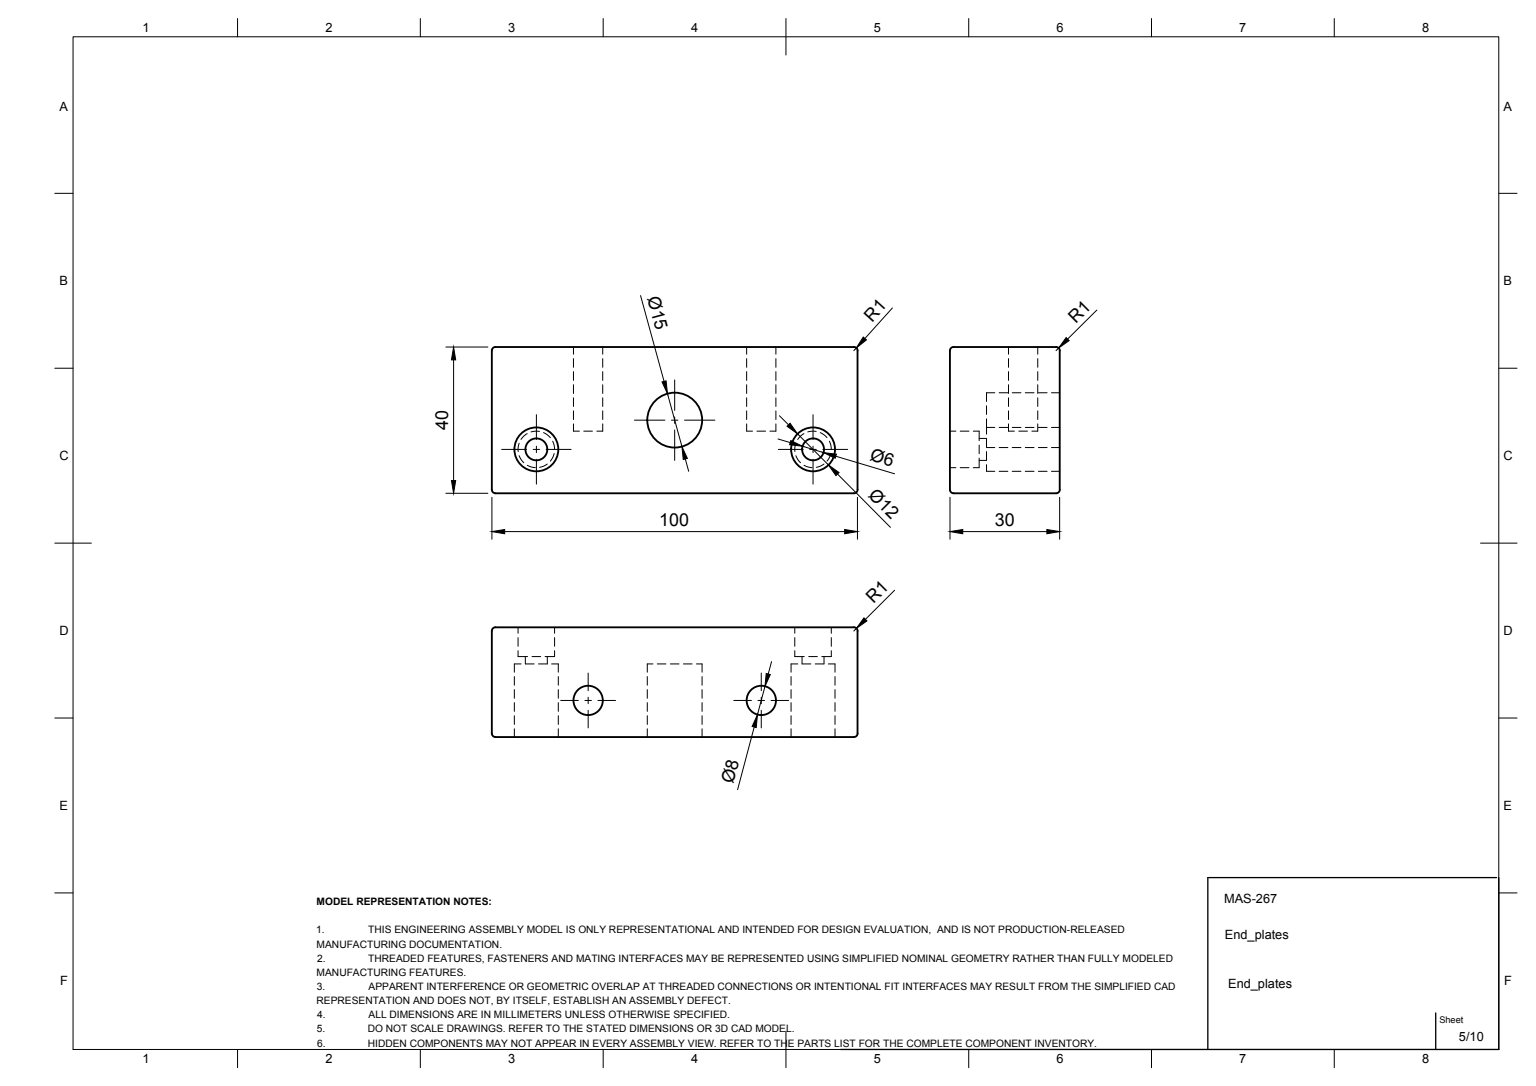
ISO-10303-21;
HEADER;
/* Generated by software containing ST-Developer
 * from STEP Tools, Inc. (www.steptools.com) 
 */

FILE_DESCRIPTION(
/* description */ (''),
/* implementation_level */ '2;1');

FILE_NAME(
/* name */ 'End_plates.step',
/* time_stamp */ '2026-10-12T15:29:24-07:00',
/* author */ (''),
/* organization */ (''),
/* preprocessor_version */ 'ST-DEVELOPER v20.2',
/* originating_system */ 'Autodesk Translation Framework v15.15.0.0',
/* authorisation */ '');

FILE_SCHEMA (('AUTOMOTIVE_DESIGN { 1 0 10303 214 3 1 1 }'));
ENDSEC;

DATA;
#10=MECHANICAL_DESIGN_GEOMETRIC_PRESENTATION_REPRESENTATION('',(#164),#9496);
#146=SHAPE_REPRESENTATION_RELATIONSHIP('SRR','None',#9540,#155);
#155=ADVANCED_BREP_SHAPE_REPRESENTATION('',(#221),#9488);
#164=STYLED_ITEM('',(#9593),#221);
#221=MANIFOLD_SOLID_BREP('Body1',#4966);
#285=SPHERICAL_SURFACE('',#5240,0.999999999999996);
#286=SPHERICAL_SURFACE('',#5244,1.00000000000001);
#287=SPHERICAL_SURFACE('',#5248,1.00000000000001);
#288=SPHERICAL_SURFACE('',#5252,0.999999999999996);
#289=SPHERICAL_SURFACE('',#5257,0.999999999999996);
#290=SPHERICAL_SURFACE('',#5261,0.999999999999996);
#291=SPHERICAL_SURFACE('',#5266,0.999999999999996);
#292=SPHERICAL_SURFACE('',#5272,1.00000000000001);
#343=FACE_BOUND('',#1011,.T.);
#344=FACE_BOUND('',#1018,.T.);
#345=FACE_BOUND('',#1021,.T.);
#346=FACE_BOUND('',#1045,.T.);
#347=FACE_BOUND('',#1046,.T.);
#348=FACE_BOUND('',#1047,.T.);
#349=FACE_BOUND('',#1050,.T.);
#350=FACE_BOUND('',#1051,.T.);
#351=FACE_BOUND('',#1054,.T.);
#352=FACE_BOUND('',#1055,.T.);
#353=FACE_BOUND('',#1059,.T.);
#498=PLANE('',#5217);
#499=PLANE('',#5222);
#500=PLANE('',#5226);
#501=PLANE('',#5230);
#502=PLANE('',#5235);
#503=PLANE('',#5284);
#504=PLANE('',#5287);
#505=PLANE('',#5288);
#506=PLANE('',#5289);
#507=PLANE('',#5290);
#508=PLANE('',#5291);
#509=PLANE('',#5294);
#510=PLANE('',#5297);
#667=FACE_OUTER_BOUND('',#1009,.T.);
#668=FACE_OUTER_BOUND('',#1010,.T.);
#669=FACE_OUTER_BOUND('',#1012,.T.);
#670=FACE_OUTER_BOUND('',#1013,.T.);
#671=FACE_OUTER_BOUND('',#1014,.T.);
#672=FACE_OUTER_BOUND('',#1015,.T.);
#673=FACE_OUTER_BOUND('',#1016,.T.);
#674=FACE_OUTER_BOUND('',#1017,.T.);
#675=FACE_OUTER_BOUND('',#1019,.T.);
#676=FACE_OUTER_BOUND('',#1020,.T.);
#677=FACE_OUTER_BOUND('',#1022,.T.);
#678=FACE_OUTER_BOUND('',#1023,.T.);
#679=FACE_OUTER_BOUND('',#1024,.T.);
#680=FACE_OUTER_BOUND('',#1025,.T.);
#681=FACE_OUTER_BOUND('',#1026,.T.);
#682=FACE_OUTER_BOUND('',#1027,.T.);
#683=FACE_OUTER_BOUND('',#1028,.T.);
#684=FACE_OUTER_BOUND('',#1029,.T.);
#685=FACE_OUTER_BOUND('',#1030,.T.);
#686=FACE_OUTER_BOUND('',#1031,.T.);
#687=FACE_OUTER_BOUND('',#1032,.T.);
#688=FACE_OUTER_BOUND('',#1033,.T.);
#689=FACE_OUTER_BOUND('',#1034,.T.);
#690=FACE_OUTER_BOUND('',#1035,.T.);
#691=FACE_OUTER_BOUND('',#1036,.T.);
#692=FACE_OUTER_BOUND('',#1037,.T.);
#693=FACE_OUTER_BOUND('',#1038,.T.);
#694=FACE_OUTER_BOUND('',#1039,.T.);
#695=FACE_OUTER_BOUND('',#1040,.T.);
#696=FACE_OUTER_BOUND('',#1041,.T.);
#697=FACE_OUTER_BOUND('',#1042,.T.);
#698=FACE_OUTER_BOUND('',#1043,.T.);
#699=FACE_OUTER_BOUND('',#1044,.T.);
#700=FACE_OUTER_BOUND('',#1048,.T.);
#701=FACE_OUTER_BOUND('',#1049,.T.);
#702=FACE_OUTER_BOUND('',#1052,.T.);
#703=FACE_OUTER_BOUND('',#1053,.T.);
#704=FACE_OUTER_BOUND('',#1056,.T.);
#705=FACE_OUTER_BOUND('',#1057,.T.);
#706=FACE_OUTER_BOUND('',#1058,.T.);
#707=FACE_OUTER_BOUND('',#1060,.T.);
#708=FACE_OUTER_BOUND('',#1061,.T.);
#1009=EDGE_LOOP('',(#3507,#3508,#3509,#3510));
#1010=EDGE_LOOP('',(#3511));
#1011=EDGE_LOOP('',(#3512));
#1012=EDGE_LOOP('',(#3513,#3514,#3515,#3516));
#1013=EDGE_LOOP('',(#3517));
#1014=EDGE_LOOP('',(#3518,#3519,#3520,#3521));
#1015=EDGE_LOOP('',(#3522));
#1016=EDGE_LOOP('',(#3523,#3524,#3525,#3526));
#1017=EDGE_LOOP('',(#3527));
#1018=EDGE_LOOP('',(#3528));
#1019=EDGE_LOOP('',(#3529,#3530,#3531,#3532));
#1020=EDGE_LOOP('',(#3533));
#1021=EDGE_LOOP('',(#3534));
#1022=EDGE_LOOP('',(#3535,#3536,#3537,#3538));
#1023=EDGE_LOOP('',(#3539,#3540,#3541,#3542));
#1024=EDGE_LOOP('',(#3543,#3544,#3545));
#1025=EDGE_LOOP('',(#3546,#3547,#3548));
#1026=EDGE_LOOP('',(#3549,#3550,#3551));
#1027=EDGE_LOOP('',(#3552,#3553,#3554));
#1028=EDGE_LOOP('',(#3555,#3556,#3557,#3558));
#1029=EDGE_LOOP('',(#3559,#3560,#3561));
#1030=EDGE_LOOP('',(#3562,#3563,#3564));
#1031=EDGE_LOOP('',(#3565,#3566,#3567,#3568));
#1032=EDGE_LOOP('',(#3569,#3570,#3571));
#1033=EDGE_LOOP('',(#3572,#3573,#3574,#3575));
#1034=EDGE_LOOP('',(#3576,#3577,#3578,#3579));
#1035=EDGE_LOOP('',(#3580,#3581,#3582));
#1036=EDGE_LOOP('',(#3583,#3584,#3585,#3586));
#1037=EDGE_LOOP('',(#3587,#3588,#3589,#3590));
#1038=EDGE_LOOP('',(#3591,#3592,#3593,#3594));
#1039=EDGE_LOOP('',(#3595,#3596,#3597,#3598));
#1040=EDGE_LOOP('',(#3599,#3600,#3601,#3602));
#1041=EDGE_LOOP('',(#3603,#3604,#3605,#3606));
#1042=EDGE_LOOP('',(#3607,#3608,#3609,#3610));
#1043=EDGE_LOOP('',(#3611,#3612,#3613,#3614));
#1044=EDGE_LOOP('',(#3615,#3616,#3617,#3618));
#1045=EDGE_LOOP('',(#3619));
#1046=EDGE_LOOP('',(#3620));
#1047=EDGE_LOOP('',(#3621));
#1048=EDGE_LOOP('',(#3622,#3623,#3624,#3625));
#1049=EDGE_LOOP('',(#3626,#3627,#3628,#3629));
#1050=EDGE_LOOP('',(#3630));
#1051=EDGE_LOOP('',(#3631));
#1052=EDGE_LOOP('',(#3632,#3633,#3634,#3635));
#1053=EDGE_LOOP('',(#3636,#3637,#3638,#3639));
#1054=EDGE_LOOP('',(#3640));
#1055=EDGE_LOOP('',(#3641));
#1056=EDGE_LOOP('',(#3642,#3643,#3644,#3645));
#1057=EDGE_LOOP('',(#3646,#3647,#3648,#3649));
#1058=EDGE_LOOP('',(#3650));
#1059=EDGE_LOOP('',(#3651));
#1060=EDGE_LOOP('',(#3652,#3653,#3654,#3655));
#1061=EDGE_LOOP('',(#3656));
#1482=LINE('',#7668,#1719);
#1483=LINE('',#7677,#1720);
#1484=LINE('',#7684,#1721);
#1485=LINE('',#7691,#1722);
#1486=LINE('',#7700,#1723);
#1487=LINE('',#7706,#1724);
#1488=LINE('',#7709,#1725);
#1489=LINE('',#7740,#1726);
#1490=LINE('',#7741,#1727);
#1491=LINE('',#7757,#1728);
#1492=LINE('',#7758,#1729);
#1493=LINE('',#7767,#1730);
#1494=LINE('',#7768,#1731);
#1495=LINE('',#7770,#1732);
#1496=LINE('',#7771,#1733);
#1497=LINE('',#7780,#1734);
#1498=LINE('',#7781,#1735);
#1499=LINE('',#7783,#1736);
#1500=LINE('',#7784,#1737);
#1501=LINE('',#7786,#1738);
#1502=LINE('',#7787,#1739);
#1503=LINE('',#7789,#1740);
#1504=LINE('',#7790,#1741);
#1505=LINE('',#7792,#1742);
#1506=LINE('',#7793,#1743);
#1507=LINE('',#7795,#1744);
#1508=LINE('',#7796,#1745);
#1509=LINE('',#7798,#1746);
#1510=LINE('',#7799,#1747);
#1511=LINE('',#7801,#1748);
#1512=LINE('',#7802,#1749);
#1513=LINE('',#7815,#1750);
#1514=LINE('',#7820,#1751);
#1719=VECTOR('',#6061,6.00000000000001);
#1720=VECTOR('',#6072,4.);
#1721=VECTOR('',#6081,4.);
#1722=VECTOR('',#6090,4.99999999999977);
#1723=VECTOR('',#6101,4.99999999999977);
#1724=VECTOR('',#6110,3.);
#1725=VECTOR('',#6113,3.);
#1726=VECTOR('',#6150,10.);
#1727=VECTOR('',#6151,10.);
#1728=VECTOR('',#6170,10.);
#1729=VECTOR('',#6171,10.);
#1730=VECTOR('',#6182,10.);
#1731=VECTOR('',#6183,10.);
#1732=VECTOR('',#6186,10.);
#1733=VECTOR('',#6187,10.);
#1734=VECTOR('',#6198,10.);
#1735=VECTOR('',#6199,10.);
#1736=VECTOR('',#6202,10.);
#1737=VECTOR('',#6203,10.);
#1738=VECTOR('',#6206,10.);
#1739=VECTOR('',#6207,10.);
#1740=VECTOR('',#6210,10.);
#1741=VECTOR('',#6211,10.);
#1742=VECTOR('',#6214,10.);
#1743=VECTOR('',#6215,10.);
#1744=VECTOR('',#6218,10.);
#1745=VECTOR('',#6219,10.);
#1746=VECTOR('',#6222,10.);
#1747=VECTOR('',#6223,10.);
#1748=VECTOR('',#6226,10.);
#1749=VECTOR('',#6227,10.);
#1750=VECTOR('',#6246,6.00000000000001);
#1751=VECTOR('',#6253,7.50000000000001);
#1951=CIRCLE('',#5215,6.00000000000001);
#1952=CIRCLE('',#5216,6.00000000000001);
#1953=CIRCLE('',#5218,3.);
#1954=CIRCLE('',#5220,4.);
#1955=CIRCLE('',#5221,4.);
#1956=CIRCLE('',#5224,4.);
#1957=CIRCLE('',#5225,4.);
#1958=CIRCLE('',#5228,4.99999999999977);
#1959=CIRCLE('',#5229,4.99999999999977);
#1960=CIRCLE('',#5231,3.);
#1961=CIRCLE('',#5233,4.99999999999977);
#1962=CIRCLE('',#5234,4.99999999999977);
#1963=CIRCLE('',#5236,3.);
#1964=CIRCLE('',#5239,3.);
#1965=CIRCLE('',#5241,0.999999999999996);
#1966=CIRCLE('',#5242,0.999999999999996);
#1967=CIRCLE('',#5243,1.);
#1968=CIRCLE('',#5245,0.999999999999996);
#1969=CIRCLE('',#5246,1.00000000000001);
#1970=CIRCLE('',#5247,1.);
#1971=CIRCLE('',#5249,0.999999999999996);
#1972=CIRCLE('',#5250,1.00000000000001);
#1973=CIRCLE('',#5251,1.);
#1974=CIRCLE('',#5253,0.999999999999996);
#1975=CIRCLE('',#5254,0.999999999999996);
#1976=CIRCLE('',#5255,1.);
#1977=CIRCLE('',#5258,0.999999999999996);
#1978=CIRCLE('',#5259,0.999999999999996);
#1979=CIRCLE('',#5260,1.);
#1980=CIRCLE('',#5262,0.999999999999996);
#1981=CIRCLE('',#5263,0.999999999999996);
#1982=CIRCLE('',#5264,1.);
#1983=CIRCLE('',#5267,0.999999999999996);
#1984=CIRCLE('',#5268,0.999999999999996);
#1985=CIRCLE('',#5269,1.);
#1986=CIRCLE('',#5273,0.999999999999996);
#1987=CIRCLE('',#5274,1.00000000000001);
#1988=CIRCLE('',#5275,1.);
#1989=CIRCLE('',#5285,7.50000000000001);
#1990=CIRCLE('',#5286,6.00000000000001);
#1991=CIRCLE('',#5293,6.00000000000001);
#1992=CIRCLE('',#5296,7.50000000000001);
#2318=VERTEX_POINT('',#7665);
#2319=VERTEX_POINT('',#7667);
#2320=VERTEX_POINT('',#7671);
#2321=VERTEX_POINT('',#7674);
#2322=VERTEX_POINT('',#7676);
#2323=VERTEX_POINT('',#7681);
#2324=VERTEX_POINT('',#7683);
#2325=VERTEX_POINT('',#7688);
#2326=VERTEX_POINT('',#7690);
#2327=VERTEX_POINT('',#7694);
#2328=VERTEX_POINT('',#7697);
#2329=VERTEX_POINT('',#7699);
#2330=VERTEX_POINT('',#7703);
#2331=VERTEX_POINT('',#7708);
#2332=VERTEX_POINT('',#7712);
#2333=VERTEX_POINT('',#7713);
#2334=VERTEX_POINT('',#7715);
#2335=VERTEX_POINT('',#7719);
#2336=VERTEX_POINT('',#7720);
#2337=VERTEX_POINT('',#7722);
#2338=VERTEX_POINT('',#7726);
#2339=VERTEX_POINT('',#7727);
#2340=VERTEX_POINT('',#7729);
#2341=VERTEX_POINT('',#7733);
#2342=VERTEX_POINT('',#7734);
#2343=VERTEX_POINT('',#7736);
#2344=VERTEX_POINT('',#7743);
#2345=VERTEX_POINT('',#7744);
#2346=VERTEX_POINT('',#7746);
#2347=VERTEX_POINT('',#7750);
#2348=VERTEX_POINT('',#7751);
#2349=VERTEX_POINT('',#7753);
#2350=VERTEX_POINT('',#7760);
#2351=VERTEX_POINT('',#7761);
#2352=VERTEX_POINT('',#7763);
#2353=VERTEX_POINT('',#7773);
#2354=VERTEX_POINT('',#7774);
#2355=VERTEX_POINT('',#7776);
#2356=VERTEX_POINT('',#7804);
#2357=VERTEX_POINT('',#7806);
#2358=VERTEX_POINT('',#7814);
#2359=VERTEX_POINT('',#7819);
#2806=EDGE_CURVE('',#2318,#2318,#1951,.T.);
#2807=EDGE_CURVE('',#2318,#2319,#1482,.T.);
#2808=EDGE_CURVE('',#2319,#2319,#1952,.T.);
#2809=EDGE_CURVE('',#2320,#2320,#1953,.T.);
#2810=EDGE_CURVE('',#2321,#2321,#1954,.T.);
#2811=EDGE_CURVE('',#2321,#2322,#1483,.T.);
#2812=EDGE_CURVE('',#2322,#2322,#1955,.T.);
#2813=EDGE_CURVE('',#2323,#2323,#1956,.T.);
#2814=EDGE_CURVE('',#2323,#2324,#1484,.T.);
#2815=EDGE_CURVE('',#2324,#2324,#1957,.T.);
#2816=EDGE_CURVE('',#2325,#2325,#1958,.T.);
#2817=EDGE_CURVE('',#2325,#2326,#1485,.T.);
#2818=EDGE_CURVE('',#2326,#2326,#1959,.T.);
#2819=EDGE_CURVE('',#2327,#2327,#1960,.T.);
#2820=EDGE_CURVE('',#2328,#2328,#1961,.T.);
#2821=EDGE_CURVE('',#2328,#2329,#1486,.T.);
#2822=EDGE_CURVE('',#2329,#2329,#1962,.T.);
#2823=EDGE_CURVE('',#2330,#2330,#1963,.T.);
#2824=EDGE_CURVE('',#2330,#2320,#1487,.T.);
#2825=EDGE_CURVE('',#2327,#2331,#1488,.T.);
#2826=EDGE_CURVE('',#2331,#2331,#1964,.T.);
#2827=EDGE_CURVE('',#2332,#2333,#1965,.F.);
#2828=EDGE_CURVE('',#2334,#2332,#1966,.F.);
#2829=EDGE_CURVE('',#2333,#2334,#1967,.F.);
#2830=EDGE_CURVE('',#2335,#2336,#1968,.F.);
#2831=EDGE_CURVE('',#2337,#2335,#1969,.F.);
#2832=EDGE_CURVE('',#2336,#2337,#1970,.F.);
#2833=EDGE_CURVE('',#2338,#2339,#1971,.F.);
#2834=EDGE_CURVE('',#2340,#2338,#1972,.F.);
#2835=EDGE_CURVE('',#2339,#2340,#1973,.F.);
#2836=EDGE_CURVE('',#2341,#2342,#1974,.F.);
#2837=EDGE_CURVE('',#2343,#2341,#1975,.F.);
#2838=EDGE_CURVE('',#2342,#2343,#1976,.F.);
#2839=EDGE_CURVE('',#2341,#2334,#1489,.T.);
#2840=EDGE_CURVE('',#2332,#2343,#1490,.T.);
#2841=EDGE_CURVE('',#2344,#2345,#1977,.F.);
#2842=EDGE_CURVE('',#2346,#2344,#1978,.F.);
#2843=EDGE_CURVE('',#2345,#2346,#1979,.F.);
#2844=EDGE_CURVE('',#2347,#2348,#1980,.F.);
#2845=EDGE_CURVE('',#2349,#2347,#1981,.F.);
#2846=EDGE_CURVE('',#2348,#2349,#1982,.F.);
#2847=EDGE_CURVE('',#2347,#2337,#1491,.T.);
#2848=EDGE_CURVE('',#2335,#2349,#1492,.T.);
#2849=EDGE_CURVE('',#2350,#2351,#1983,.F.);
#2850=EDGE_CURVE('',#2352,#2350,#1984,.F.);
#2851=EDGE_CURVE('',#2351,#2352,#1985,.F.);
#2852=EDGE_CURVE('',#2350,#2340,#1493,.T.);
#2853=EDGE_CURVE('',#2338,#2352,#1494,.T.);
#2854=EDGE_CURVE('',#2342,#2351,#1495,.T.);
#2855=EDGE_CURVE('',#2352,#2341,#1496,.T.);
#2856=EDGE_CURVE('',#2353,#2354,#1986,.F.);
#2857=EDGE_CURVE('',#2355,#2353,#1987,.F.);
#2858=EDGE_CURVE('',#2354,#2355,#1988,.F.);
#2859=EDGE_CURVE('',#2344,#2355,#1497,.T.);
#2860=EDGE_CURVE('',#2353,#2346,#1498,.T.);
#2861=EDGE_CURVE('',#2351,#2354,#1499,.T.);
#2862=EDGE_CURVE('',#2355,#2350,#1500,.T.);
#2863=EDGE_CURVE('',#2354,#2348,#1501,.T.);
#2864=EDGE_CURVE('',#2349,#2353,#1502,.T.);
#2865=EDGE_CURVE('',#2348,#2342,#1503,.T.);
#2866=EDGE_CURVE('',#2343,#2347,#1504,.T.);
#2867=EDGE_CURVE('',#2336,#2345,#1505,.T.);
#2868=EDGE_CURVE('',#2346,#2335,#1506,.T.);
#2869=EDGE_CURVE('',#2345,#2339,#1507,.T.);
#2870=EDGE_CURVE('',#2340,#2344,#1508,.T.);
#2871=EDGE_CURVE('',#2339,#2333,#1509,.T.);
#2872=EDGE_CURVE('',#2334,#2338,#1510,.T.);
#2873=EDGE_CURVE('',#2333,#2336,#1511,.T.);
#2874=EDGE_CURVE('',#2337,#2332,#1512,.T.);
#2875=EDGE_CURVE('',#2356,#2356,#1989,.T.);
#2876=EDGE_CURVE('',#2357,#2357,#1990,.T.);
#2877=EDGE_CURVE('',#2357,#2358,#1513,.T.);
#2878=EDGE_CURVE('',#2358,#2358,#1991,.T.);
#2879=EDGE_CURVE('',#2356,#2359,#1514,.T.);
#2880=EDGE_CURVE('',#2359,#2359,#1992,.T.);
#3507=ORIENTED_EDGE('',*,*,#2806,.T.);
#3508=ORIENTED_EDGE('',*,*,#2807,.T.);
#3509=ORIENTED_EDGE('',*,*,#2808,.F.);
#3510=ORIENTED_EDGE('',*,*,#2807,.F.);
#3511=ORIENTED_EDGE('',*,*,#2806,.F.);
#3512=ORIENTED_EDGE('',*,*,#2809,.F.);
#3513=ORIENTED_EDGE('',*,*,#2810,.F.);
#3514=ORIENTED_EDGE('',*,*,#2811,.T.);
#3515=ORIENTED_EDGE('',*,*,#2812,.T.);
#3516=ORIENTED_EDGE('',*,*,#2811,.F.);
#3517=ORIENTED_EDGE('',*,*,#2812,.F.);
#3518=ORIENTED_EDGE('',*,*,#2813,.F.);
#3519=ORIENTED_EDGE('',*,*,#2814,.T.);
#3520=ORIENTED_EDGE('',*,*,#2815,.T.);
#3521=ORIENTED_EDGE('',*,*,#2814,.F.);
#3522=ORIENTED_EDGE('',*,*,#2815,.F.);
#3523=ORIENTED_EDGE('',*,*,#2816,.F.);
#3524=ORIENTED_EDGE('',*,*,#2817,.T.);
#3525=ORIENTED_EDGE('',*,*,#2818,.T.);
#3526=ORIENTED_EDGE('',*,*,#2817,.F.);
#3527=ORIENTED_EDGE('',*,*,#2818,.F.);
#3528=ORIENTED_EDGE('',*,*,#2819,.F.);
#3529=ORIENTED_EDGE('',*,*,#2820,.F.);
#3530=ORIENTED_EDGE('',*,*,#2821,.T.);
#3531=ORIENTED_EDGE('',*,*,#2822,.T.);
#3532=ORIENTED_EDGE('',*,*,#2821,.F.);
#3533=ORIENTED_EDGE('',*,*,#2822,.F.);
#3534=ORIENTED_EDGE('',*,*,#2823,.F.);
#3535=ORIENTED_EDGE('',*,*,#2823,.T.);
#3536=ORIENTED_EDGE('',*,*,#2824,.T.);
#3537=ORIENTED_EDGE('',*,*,#2809,.T.);
#3538=ORIENTED_EDGE('',*,*,#2824,.F.);
#3539=ORIENTED_EDGE('',*,*,#2819,.T.);
#3540=ORIENTED_EDGE('',*,*,#2825,.T.);
#3541=ORIENTED_EDGE('',*,*,#2826,.F.);
#3542=ORIENTED_EDGE('',*,*,#2825,.F.);
#3543=ORIENTED_EDGE('',*,*,#2827,.F.);
#3544=ORIENTED_EDGE('',*,*,#2828,.F.);
#3545=ORIENTED_EDGE('',*,*,#2829,.F.);
#3546=ORIENTED_EDGE('',*,*,#2830,.F.);
#3547=ORIENTED_EDGE('',*,*,#2831,.F.);
#3548=ORIENTED_EDGE('',*,*,#2832,.F.);
#3549=ORIENTED_EDGE('',*,*,#2833,.F.);
#3550=ORIENTED_EDGE('',*,*,#2834,.F.);
#3551=ORIENTED_EDGE('',*,*,#2835,.F.);
#3552=ORIENTED_EDGE('',*,*,#2836,.F.);
#3553=ORIENTED_EDGE('',*,*,#2837,.F.);
#3554=ORIENTED_EDGE('',*,*,#2838,.F.);
#3555=ORIENTED_EDGE('',*,*,#2837,.T.);
#3556=ORIENTED_EDGE('',*,*,#2839,.T.);
#3557=ORIENTED_EDGE('',*,*,#2828,.T.);
#3558=ORIENTED_EDGE('',*,*,#2840,.T.);
#3559=ORIENTED_EDGE('',*,*,#2841,.F.);
#3560=ORIENTED_EDGE('',*,*,#2842,.F.);
#3561=ORIENTED_EDGE('',*,*,#2843,.F.);
#3562=ORIENTED_EDGE('',*,*,#2844,.F.);
#3563=ORIENTED_EDGE('',*,*,#2845,.F.);
#3564=ORIENTED_EDGE('',*,*,#2846,.F.);
#3565=ORIENTED_EDGE('',*,*,#2845,.T.);
#3566=ORIENTED_EDGE('',*,*,#2847,.T.);
#3567=ORIENTED_EDGE('',*,*,#2831,.T.);
#3568=ORIENTED_EDGE('',*,*,#2848,.T.);
#3569=ORIENTED_EDGE('',*,*,#2849,.F.);
#3570=ORIENTED_EDGE('',*,*,#2850,.F.);
#3571=ORIENTED_EDGE('',*,*,#2851,.F.);
#3572=ORIENTED_EDGE('',*,*,#2850,.T.);
#3573=ORIENTED_EDGE('',*,*,#2852,.T.);
#3574=ORIENTED_EDGE('',*,*,#2834,.T.);
#3575=ORIENTED_EDGE('',*,*,#2853,.T.);
#3576=ORIENTED_EDGE('',*,*,#2836,.T.);
#3577=ORIENTED_EDGE('',*,*,#2854,.T.);
#3578=ORIENTED_EDGE('',*,*,#2851,.T.);
#3579=ORIENTED_EDGE('',*,*,#2855,.T.);
#3580=ORIENTED_EDGE('',*,*,#2856,.F.);
#3581=ORIENTED_EDGE('',*,*,#2857,.F.);
#3582=ORIENTED_EDGE('',*,*,#2858,.F.);
#3583=ORIENTED_EDGE('',*,*,#2842,.T.);
#3584=ORIENTED_EDGE('',*,*,#2859,.T.);
#3585=ORIENTED_EDGE('',*,*,#2857,.T.);
#3586=ORIENTED_EDGE('',*,*,#2860,.T.);
#3587=ORIENTED_EDGE('',*,*,#2849,.T.);
#3588=ORIENTED_EDGE('',*,*,#2861,.T.);
#3589=ORIENTED_EDGE('',*,*,#2858,.T.);
#3590=ORIENTED_EDGE('',*,*,#2862,.T.);
#3591=ORIENTED_EDGE('',*,*,#2856,.T.);
#3592=ORIENTED_EDGE('',*,*,#2863,.T.);
#3593=ORIENTED_EDGE('',*,*,#2846,.T.);
#3594=ORIENTED_EDGE('',*,*,#2864,.T.);
#3595=ORIENTED_EDGE('',*,*,#2844,.T.);
#3596=ORIENTED_EDGE('',*,*,#2865,.T.);
#3597=ORIENTED_EDGE('',*,*,#2838,.T.);
#3598=ORIENTED_EDGE('',*,*,#2866,.T.);
#3599=ORIENTED_EDGE('',*,*,#2830,.T.);
#3600=ORIENTED_EDGE('',*,*,#2867,.T.);
#3601=ORIENTED_EDGE('',*,*,#2843,.T.);
#3602=ORIENTED_EDGE('',*,*,#2868,.T.);
#3603=ORIENTED_EDGE('',*,*,#2841,.T.);
#3604=ORIENTED_EDGE('',*,*,#2869,.T.);
#3605=ORIENTED_EDGE('',*,*,#2835,.T.);
#3606=ORIENTED_EDGE('',*,*,#2870,.T.);
#3607=ORIENTED_EDGE('',*,*,#2833,.T.);
#3608=ORIENTED_EDGE('',*,*,#2871,.T.);
#3609=ORIENTED_EDGE('',*,*,#2829,.T.);
#3610=ORIENTED_EDGE('',*,*,#2872,.T.);
#3611=ORIENTED_EDGE('',*,*,#2827,.T.);
#3612=ORIENTED_EDGE('',*,*,#2873,.T.);
#3613=ORIENTED_EDGE('',*,*,#2832,.T.);
#3614=ORIENTED_EDGE('',*,*,#2874,.T.);
#3615=ORIENTED_EDGE('',*,*,#2847,.F.);
#3616=ORIENTED_EDGE('',*,*,#2866,.F.);
#3617=ORIENTED_EDGE('',*,*,#2840,.F.);
#3618=ORIENTED_EDGE('',*,*,#2874,.F.);
#3619=ORIENTED_EDGE('',*,*,#2808,.T.);
#3620=ORIENTED_EDGE('',*,*,#2875,.T.);
#3621=ORIENTED_EDGE('',*,*,#2876,.T.);
#3622=ORIENTED_EDGE('',*,*,#2853,.F.);
#3623=ORIENTED_EDGE('',*,*,#2872,.F.);
#3624=ORIENTED_EDGE('',*,*,#2839,.F.);
#3625=ORIENTED_EDGE('',*,*,#2855,.F.);
#3626=ORIENTED_EDGE('',*,*,#2854,.F.);
#3627=ORIENTED_EDGE('',*,*,#2865,.F.);
#3628=ORIENTED_EDGE('',*,*,#2863,.F.);
#3629=ORIENTED_EDGE('',*,*,#2861,.F.);
#3630=ORIENTED_EDGE('',*,*,#2810,.T.);
#3631=ORIENTED_EDGE('',*,*,#2813,.T.);
#3632=ORIENTED_EDGE('',*,*,#2860,.F.);
#3633=ORIENTED_EDGE('',*,*,#2864,.F.);
#3634=ORIENTED_EDGE('',*,*,#2848,.F.);
#3635=ORIENTED_EDGE('',*,*,#2868,.F.);
#3636=ORIENTED_EDGE('',*,*,#2859,.F.);
#3637=ORIENTED_EDGE('',*,*,#2870,.F.);
#3638=ORIENTED_EDGE('',*,*,#2852,.F.);
#3639=ORIENTED_EDGE('',*,*,#2862,.F.);
#3640=ORIENTED_EDGE('',*,*,#2816,.T.);
#3641=ORIENTED_EDGE('',*,*,#2820,.T.);
#3642=ORIENTED_EDGE('',*,*,#2867,.F.);
#3643=ORIENTED_EDGE('',*,*,#2873,.F.);
#3644=ORIENTED_EDGE('',*,*,#2871,.F.);
#3645=ORIENTED_EDGE('',*,*,#2869,.F.);
#3646=ORIENTED_EDGE('',*,*,#2876,.F.);
#3647=ORIENTED_EDGE('',*,*,#2877,.T.);
#3648=ORIENTED_EDGE('',*,*,#2878,.T.);
#3649=ORIENTED_EDGE('',*,*,#2877,.F.);
#3650=ORIENTED_EDGE('',*,*,#2878,.F.);
#3651=ORIENTED_EDGE('',*,*,#2826,.T.);
#3652=ORIENTED_EDGE('',*,*,#2875,.F.);
#3653=ORIENTED_EDGE('',*,*,#2879,.T.);
#3654=ORIENTED_EDGE('',*,*,#2880,.T.);
#3655=ORIENTED_EDGE('',*,*,#2879,.F.);
#3656=ORIENTED_EDGE('',*,*,#2880,.F.);
#4568=CYLINDRICAL_SURFACE('',#5214,6.00000000000001);
#4569=CYLINDRICAL_SURFACE('',#5219,4.);
#4570=CYLINDRICAL_SURFACE('',#5223,4.);
#4571=CYLINDRICAL_SURFACE('',#5227,4.99999999999977);
#4572=CYLINDRICAL_SURFACE('',#5232,4.99999999999977);
#4573=CYLINDRICAL_SURFACE('',#5237,3.);
#4574=CYLINDRICAL_SURFACE('',#5238,3.);
#4575=CYLINDRICAL_SURFACE('',#5256,1.);
#4576=CYLINDRICAL_SURFACE('',#5265,1.);
#4577=CYLINDRICAL_SURFACE('',#5270,1.);
#4578=CYLINDRICAL_SURFACE('',#5271,1.);
#4579=CYLINDRICAL_SURFACE('',#5276,1.);
#4580=CYLINDRICAL_SURFACE('',#5277,1.);
#4581=CYLINDRICAL_SURFACE('',#5278,1.);
#4582=CYLINDRICAL_SURFACE('',#5279,1.);
#4583=CYLINDRICAL_SURFACE('',#5280,1.);
#4584=CYLINDRICAL_SURFACE('',#5281,1.);
#4585=CYLINDRICAL_SURFACE('',#5282,1.);
#4586=CYLINDRICAL_SURFACE('',#5283,1.);
#4587=CYLINDRICAL_SURFACE('',#5292,6.00000000000001);
#4588=CYLINDRICAL_SURFACE('',#5295,7.50000000000001);
#4678=ADVANCED_FACE('',(#667),#4568,.F.);
#4679=ADVANCED_FACE('',(#668,#343),#498,.F.);
#4680=ADVANCED_FACE('',(#669),#4569,.F.);
#4681=ADVANCED_FACE('',(#670),#499,.T.);
#4682=ADVANCED_FACE('',(#671),#4570,.F.);
#4683=ADVANCED_FACE('',(#672),#500,.T.);
#4684=ADVANCED_FACE('',(#673),#4571,.F.);
#4685=ADVANCED_FACE('',(#674,#344),#501,.T.);
#4686=ADVANCED_FACE('',(#675),#4572,.F.);
#4687=ADVANCED_FACE('',(#676,#345),#502,.T.);
#4688=ADVANCED_FACE('',(#677),#4573,.F.);
#4689=ADVANCED_FACE('',(#678),#4574,.F.);
#4690=ADVANCED_FACE('',(#679),#285,.T.);
#4691=ADVANCED_FACE('',(#680),#286,.T.);
#4692=ADVANCED_FACE('',(#681),#287,.T.);
#4693=ADVANCED_FACE('',(#682),#288,.T.);
#4694=ADVANCED_FACE('',(#683),#4575,.T.);
#4695=ADVANCED_FACE('',(#684),#289,.T.);
#4696=ADVANCED_FACE('',(#685),#290,.T.);
#4697=ADVANCED_FACE('',(#686),#4576,.T.);
#4698=ADVANCED_FACE('',(#687),#291,.T.);
#4699=ADVANCED_FACE('',(#688),#4577,.T.);
#4700=ADVANCED_FACE('',(#689),#4578,.T.);
#4701=ADVANCED_FACE('',(#690),#292,.T.);
#4702=ADVANCED_FACE('',(#691),#4579,.T.);
#4703=ADVANCED_FACE('',(#692),#4580,.T.);
#4704=ADVANCED_FACE('',(#693),#4581,.T.);
#4705=ADVANCED_FACE('',(#694),#4582,.T.);
#4706=ADVANCED_FACE('',(#695),#4583,.T.);
#4707=ADVANCED_FACE('',(#696),#4584,.T.);
#4708=ADVANCED_FACE('',(#697),#4585,.T.);
#4709=ADVANCED_FACE('',(#698),#4586,.T.);
#4710=ADVANCED_FACE('',(#699,#346,#347,#348),#503,.T.);
#4711=ADVANCED_FACE('',(#700),#504,.T.);
#4712=ADVANCED_FACE('',(#701,#349,#350),#505,.T.);
#4713=ADVANCED_FACE('',(#702),#506,.T.);
#4714=ADVANCED_FACE('',(#703,#351,#352),#507,.T.);
#4715=ADVANCED_FACE('',(#704),#508,.T.);
#4716=ADVANCED_FACE('',(#705),#4587,.F.);
#4717=ADVANCED_FACE('',(#706,#353),#509,.F.);
#4718=ADVANCED_FACE('',(#707),#4588,.F.);
#4719=ADVANCED_FACE('',(#708),#510,.F.);
#4966=CLOSED_SHELL('',(#4678,#4679,#4680,#4681,#4682,#4683,#4684,#4685,
#4686,#4687,#4688,#4689,#4690,#4691,#4692,#4693,#4694,#4695,#4696,#4697,
#4698,#4699,#4700,#4701,#4702,#4703,#4704,#4705,#4706,#4707,#4708,#4709,
#4710,#4711,#4712,#4713,#4714,#4715,#4716,#4717,#4718,#4719));
#5213=AXIS2_PLACEMENT_3D('',#7663,#6055,#6056);
#5214=AXIS2_PLACEMENT_3D('',#7664,#6057,#6058);
#5215=AXIS2_PLACEMENT_3D('',#7666,#6059,#6060);
#5216=AXIS2_PLACEMENT_3D('',#7669,#6062,#6063);
#5217=AXIS2_PLACEMENT_3D('',#7670,#6064,#6065);
#5218=AXIS2_PLACEMENT_3D('',#7672,#6066,#6067);
#5219=AXIS2_PLACEMENT_3D('',#7673,#6068,#6069);
#5220=AXIS2_PLACEMENT_3D('',#7675,#6070,#6071);
#5221=AXIS2_PLACEMENT_3D('',#7678,#6073,#6074);
#5222=AXIS2_PLACEMENT_3D('',#7679,#6075,#6076);
#5223=AXIS2_PLACEMENT_3D('',#7680,#6077,#6078);
#5224=AXIS2_PLACEMENT_3D('',#7682,#6079,#6080);
#5225=AXIS2_PLACEMENT_3D('',#7685,#6082,#6083);
#5226=AXIS2_PLACEMENT_3D('',#7686,#6084,#6085);
#5227=AXIS2_PLACEMENT_3D('',#7687,#6086,#6087);
#5228=AXIS2_PLACEMENT_3D('',#7689,#6088,#6089);
#5229=AXIS2_PLACEMENT_3D('',#7692,#6091,#6092);
#5230=AXIS2_PLACEMENT_3D('',#7693,#6093,#6094);
#5231=AXIS2_PLACEMENT_3D('',#7695,#6095,#6096);
#5232=AXIS2_PLACEMENT_3D('',#7696,#6097,#6098);
#5233=AXIS2_PLACEMENT_3D('',#7698,#6099,#6100);
#5234=AXIS2_PLACEMENT_3D('',#7701,#6102,#6103);
#5235=AXIS2_PLACEMENT_3D('',#7702,#6104,#6105);
#5236=AXIS2_PLACEMENT_3D('',#7704,#6106,#6107);
#5237=AXIS2_PLACEMENT_3D('',#7705,#6108,#6109);
#5238=AXIS2_PLACEMENT_3D('',#7707,#6111,#6112);
#5239=AXIS2_PLACEMENT_3D('',#7710,#6114,#6115);
#5240=AXIS2_PLACEMENT_3D('',#7711,#6116,#6117);
#5241=AXIS2_PLACEMENT_3D('',#7714,#6118,#6119);
#5242=AXIS2_PLACEMENT_3D('',#7716,#6120,#6121);
#5243=AXIS2_PLACEMENT_3D('',#7717,#6122,#6123);
#5244=AXIS2_PLACEMENT_3D('',#7718,#6124,#6125);
#5245=AXIS2_PLACEMENT_3D('',#7721,#6126,#6127);
#5246=AXIS2_PLACEMENT_3D('',#7723,#6128,#6129);
#5247=AXIS2_PLACEMENT_3D('',#7724,#6130,#6131);
#5248=AXIS2_PLACEMENT_3D('',#7725,#6132,#6133);
#5249=AXIS2_PLACEMENT_3D('',#7728,#6134,#6135);
#5250=AXIS2_PLACEMENT_3D('',#7730,#6136,#6137);
#5251=AXIS2_PLACEMENT_3D('',#7731,#6138,#6139);
#5252=AXIS2_PLACEMENT_3D('',#7732,#6140,#6141);
#5253=AXIS2_PLACEMENT_3D('',#7735,#6142,#6143);
#5254=AXIS2_PLACEMENT_3D('',#7737,#6144,#6145);
#5255=AXIS2_PLACEMENT_3D('',#7738,#6146,#6147);
#5256=AXIS2_PLACEMENT_3D('',#7739,#6148,#6149);
#5257=AXIS2_PLACEMENT_3D('',#7742,#6152,#6153);
#5258=AXIS2_PLACEMENT_3D('',#7745,#6154,#6155);
#5259=AXIS2_PLACEMENT_3D('',#7747,#6156,#6157);
#5260=AXIS2_PLACEMENT_3D('',#7748,#6158,#6159);
#5261=AXIS2_PLACEMENT_3D('',#7749,#6160,#6161);
#5262=AXIS2_PLACEMENT_3D('',#7752,#6162,#6163);
#5263=AXIS2_PLACEMENT_3D('',#7754,#6164,#6165);
#5264=AXIS2_PLACEMENT_3D('',#7755,#6166,#6167);
#5265=AXIS2_PLACEMENT_3D('',#7756,#6168,#6169);
#5266=AXIS2_PLACEMENT_3D('',#7759,#6172,#6173);
#5267=AXIS2_PLACEMENT_3D('',#7762,#6174,#6175);
#5268=AXIS2_PLACEMENT_3D('',#7764,#6176,#6177);
#5269=AXIS2_PLACEMENT_3D('',#7765,#6178,#6179);
#5270=AXIS2_PLACEMENT_3D('',#7766,#6180,#6181);
#5271=AXIS2_PLACEMENT_3D('',#7769,#6184,#6185);
#5272=AXIS2_PLACEMENT_3D('',#7772,#6188,#6189);
#5273=AXIS2_PLACEMENT_3D('',#7775,#6190,#6191);
#5274=AXIS2_PLACEMENT_3D('',#7777,#6192,#6193);
#5275=AXIS2_PLACEMENT_3D('',#7778,#6194,#6195);
#5276=AXIS2_PLACEMENT_3D('',#7779,#6196,#6197);
#5277=AXIS2_PLACEMENT_3D('',#7782,#6200,#6201);
#5278=AXIS2_PLACEMENT_3D('',#7785,#6204,#6205);
#5279=AXIS2_PLACEMENT_3D('',#7788,#6208,#6209);
#5280=AXIS2_PLACEMENT_3D('',#7791,#6212,#6213);
#5281=AXIS2_PLACEMENT_3D('',#7794,#6216,#6217);
#5282=AXIS2_PLACEMENT_3D('',#7797,#6220,#6221);
#5283=AXIS2_PLACEMENT_3D('',#7800,#6224,#6225);
#5284=AXIS2_PLACEMENT_3D('',#7803,#6228,#6229);
#5285=AXIS2_PLACEMENT_3D('',#7805,#6230,#6231);
#5286=AXIS2_PLACEMENT_3D('',#7807,#6232,#6233);
#5287=AXIS2_PLACEMENT_3D('',#7808,#6234,#6235);
#5288=AXIS2_PLACEMENT_3D('',#7809,#6236,#6237);
#5289=AXIS2_PLACEMENT_3D('',#7810,#6238,#6239);
#5290=AXIS2_PLACEMENT_3D('',#7811,#6240,#6241);
#5291=AXIS2_PLACEMENT_3D('',#7812,#6242,#6243);
#5292=AXIS2_PLACEMENT_3D('',#7813,#6244,#6245);
#5293=AXIS2_PLACEMENT_3D('',#7816,#6247,#6248);
#5294=AXIS2_PLACEMENT_3D('',#7817,#6249,#6250);
#5295=AXIS2_PLACEMENT_3D('',#7818,#6251,#6252);
#5296=AXIS2_PLACEMENT_3D('',#7821,#6254,#6255);
#5297=AXIS2_PLACEMENT_3D('',#7822,#6256,#6257);
#6055=DIRECTION('axis',(0.,0.,1.));
#6056=DIRECTION('refdir',(1.,0.,0.));
#6057=DIRECTION('center_axis',(-1.,0.,0.));
#6058=DIRECTION('ref_axis',(0.,1.,0.));
#6059=DIRECTION('center_axis',(1.,0.,0.));
#6060=DIRECTION('ref_axis',(0.,1.,0.));
#6061=DIRECTION('',(-1.,0.,0.));
#6062=DIRECTION('center_axis',(1.,0.,0.));
#6063=DIRECTION('ref_axis',(0.,1.,0.));
#6064=DIRECTION('center_axis',(1.,0.,0.));
#6065=DIRECTION('ref_axis',(0.,1.,0.));
#6066=DIRECTION('center_axis',(-1.,0.,0.));
#6067=DIRECTION('ref_axis',(0.,1.,0.));
#6068=DIRECTION('center_axis',(0.,0.,-1.));
#6069=DIRECTION('ref_axis',(1.,0.,0.));
#6070=DIRECTION('center_axis',(0.,0.,-1.));
#6071=DIRECTION('ref_axis',(1.,0.,0.));
#6072=DIRECTION('',(0.,0.,-1.));
#6073=DIRECTION('center_axis',(0.,0.,-1.));
#6074=DIRECTION('ref_axis',(1.,0.,0.));
#6075=DIRECTION('center_axis',(0.,0.,1.));
#6076=DIRECTION('ref_axis',(1.,0.,0.));
#6077=DIRECTION('center_axis',(0.,0.,-1.));
#6078=DIRECTION('ref_axis',(1.,0.,0.));
#6079=DIRECTION('center_axis',(0.,0.,-1.));
#6080=DIRECTION('ref_axis',(1.,0.,0.));
#6081=DIRECTION('',(0.,0.,-1.));
#6082=DIRECTION('center_axis',(0.,0.,-1.));
#6083=DIRECTION('ref_axis',(1.,0.,0.));
#6084=DIRECTION('center_axis',(0.,0.,1.));
#6085=DIRECTION('ref_axis',(1.,0.,0.));
#6086=DIRECTION('center_axis',(-1.,0.,0.));
#6087=DIRECTION('ref_axis',(0.,1.,0.));
#6088=DIRECTION('center_axis',(-1.,0.,0.));
#6089=DIRECTION('ref_axis',(0.,1.,0.));
#6090=DIRECTION('',(-1.,0.,0.));
#6091=DIRECTION('center_axis',(-1.,0.,0.));
#6092=DIRECTION('ref_axis',(0.,1.,0.));
#6093=DIRECTION('center_axis',(1.,0.,0.));
#6094=DIRECTION('ref_axis',(0.,1.,0.));
#6095=DIRECTION('center_axis',(1.,0.,0.));
#6096=DIRECTION('ref_axis',(0.,1.,0.));
#6097=DIRECTION('center_axis',(-1.,0.,0.));
#6098=DIRECTION('ref_axis',(0.,1.,0.));
#6099=DIRECTION('center_axis',(-1.,0.,0.));
#6100=DIRECTION('ref_axis',(0.,1.,0.));
#6101=DIRECTION('',(-1.,0.,0.));
#6102=DIRECTION('center_axis',(-1.,0.,0.));
#6103=DIRECTION('ref_axis',(0.,1.,0.));
#6104=DIRECTION('center_axis',(1.,0.,0.));
#6105=DIRECTION('ref_axis',(0.,1.,0.));
#6106=DIRECTION('center_axis',(1.,0.,0.));
#6107=DIRECTION('ref_axis',(0.,1.,0.));
#6108=DIRECTION('center_axis',(-1.,0.,0.));
#6109=DIRECTION('ref_axis',(0.,1.,0.));
#6110=DIRECTION('',(-1.,0.,0.));
#6111=DIRECTION('center_axis',(-1.,0.,0.));
#6112=DIRECTION('ref_axis',(0.,1.,0.));
#6113=DIRECTION('',(-1.,0.,0.));
#6114=DIRECTION('center_axis',(1.,0.,0.));
#6115=DIRECTION('ref_axis',(0.,1.,0.));
#6116=DIRECTION('center_axis',(-0.40824829046386,-0.816496580927727,-0.408248290463864));
#6117=DIRECTION('ref_axis',(-0.577350269189625,0.577350269189625,-0.577350269189628));
#6118=DIRECTION('center_axis',(0.,1.,0.));
#6119=DIRECTION('ref_axis',(-1.,0.,0.));
#6120=DIRECTION('center_axis',(0.,0.,-1.));
#6121=DIRECTION('ref_axis',(0.,1.,0.));
#6122=DIRECTION('center_axis',(-1.,0.,0.));
#6123=DIRECTION('ref_axis',(0.,0.,-1.));
#6124=DIRECTION('center_axis',(0.408248290463869,0.408248290463855,-0.816496580927727));
#6125=DIRECTION('ref_axis',(-0.577350269189633,-0.577350269189619,-0.577350269189626));
#6126=DIRECTION('center_axis',(-1.,0.,1.77635683940025E-14));
#6127=DIRECTION('ref_axis',(0.,-1.,0.));
#6128=DIRECTION('center_axis',(0.,0.,-1.));
#6129=DIRECTION('ref_axis',(-1.,0.,0.));
#6130=DIRECTION('center_axis',(0.,-1.,0.));
#6131=DIRECTION('ref_axis',(0.,0.,-1.));
#6132=DIRECTION('center_axis',(-0.408248290463856,-0.408248290463856,-0.816496580927733));
#6133=DIRECTION('ref_axis',(0.577350269189645,0.577350269189616,-0.577350269189616));
#6134=DIRECTION('center_axis',(1.,0.,1.77635683940025E-14));
#6135=DIRECTION('ref_axis',(0.,1.,0.));
#6136=DIRECTION('center_axis',(0.,0.,-1.));
#6137=DIRECTION('ref_axis',(1.,0.,0.));
#6138=DIRECTION('center_axis',(0.,1.,0.));
#6139=DIRECTION('ref_axis',(0.,0.,-1.));
#6140=DIRECTION('center_axis',(-0.40824829046386,-0.816496580927727,0.408248290463864));
#6141=DIRECTION('ref_axis',(-0.577350269189625,0.577350269189625,0.577350269189628));
#6142=DIRECTION('center_axis',(-1.,0.,0.));
#6143=DIRECTION('ref_axis',(0.,1.,0.));
#6144=DIRECTION('center_axis',(0.,0.,1.));
#6145=DIRECTION('ref_axis',(-1.,0.,0.));
#6146=DIRECTION('center_axis',(0.,1.,0.));
#6147=DIRECTION('ref_axis',(0.,0.,1.));
#6148=DIRECTION('center_axis',(0.,0.,1.));
#6149=DIRECTION('ref_axis',(-0.707106781186541,0.707106781186554,0.));
#6150=DIRECTION('',(0.,0.,-1.));
#6151=DIRECTION('',(0.,0.,1.));
#6152=DIRECTION('center_axis',(-0.408248290463862,0.408248290463855,-0.816496580927731));
#6153=DIRECTION('ref_axis',(0.577350269189628,-0.577350269189628,-0.577350269189621));
#6154=DIRECTION('center_axis',(0.,-1.,0.));
#6155=DIRECTION('ref_axis',(1.,0.,0.));
#6156=DIRECTION('center_axis',(0.,0.,-1.));
#6157=DIRECTION('ref_axis',(0.,-1.,0.));
#6158=DIRECTION('center_axis',(1.,-1.77635683940026E-14,0.));
#6159=DIRECTION('ref_axis',(0.,0.,-1.));
#6160=DIRECTION('center_axis',(-0.408248290463862,-0.408248290463855,-0.816496580927731));
#6161=DIRECTION('ref_axis',(-0.57735026918964,-0.577350269189619,0.577350269189619));
#6162=DIRECTION('center_axis',(0.,-1.,0.));
#6163=DIRECTION('ref_axis',(-1.,0.,0.));
#6164=DIRECTION('center_axis',(0.,0.,1.));
#6165=DIRECTION('ref_axis',(0.,-1.,0.));
#6166=DIRECTION('center_axis',(-1.,-1.77635683940026E-14,0.));
#6167=DIRECTION('ref_axis',(0.,0.,1.));
#6168=DIRECTION('center_axis',(0.,0.,1.));
#6169=DIRECTION('ref_axis',(-0.707106781186554,-0.707106781186541,0.));
#6170=DIRECTION('',(0.,0.,-1.));
#6171=DIRECTION('',(0.,0.,1.));
#6172=DIRECTION('center_axis',(0.408248290463862,0.408248290463855,-0.816496580927731));
#6173=DIRECTION('ref_axis',(0.577350269189628,0.577350269189628,0.577350269189621));
#6174=DIRECTION('center_axis',(0.,1.,0.));
#6175=DIRECTION('ref_axis',(1.,0.,0.));
#6176=DIRECTION('center_axis',(0.,0.,1.));
#6177=DIRECTION('ref_axis',(0.,1.,0.));
#6178=DIRECTION('center_axis',(1.,1.77635683940026E-14,0.));
#6179=DIRECTION('ref_axis',(0.,0.,1.));
#6180=DIRECTION('center_axis',(0.,0.,1.));
#6181=DIRECTION('ref_axis',(0.707106781186554,0.707106781186541,0.));
#6182=DIRECTION('',(0.,0.,-1.));
#6183=DIRECTION('',(0.,0.,1.));
#6184=DIRECTION('center_axis',(-1.,0.,0.));
#6185=DIRECTION('ref_axis',(0.,0.707106781186546,0.707106781186549));
#6186=DIRECTION('',(1.,0.,0.));
#6187=DIRECTION('',(-1.,0.,0.));
#6188=DIRECTION('center_axis',(0.408248290463856,-0.408248290463856,-0.816496580927733));
#6189=DIRECTION('ref_axis',(0.577350269189645,-0.577350269189616,0.577350269189616));
#6190=DIRECTION('center_axis',(1.,0.,-1.77635683940025E-14));
#6191=DIRECTION('ref_axis',(0.,-1.,0.));
#6192=DIRECTION('center_axis',(0.,0.,1.));
#6193=DIRECTION('ref_axis',(1.,0.,0.));
#6194=DIRECTION('center_axis',(0.,-1.,0.));
#6195=DIRECTION('ref_axis',(0.,0.,1.));
#6196=DIRECTION('center_axis',(0.,0.,-1.));
#6197=DIRECTION('ref_axis',(0.707106781186554,-0.707106781186541,0.));
#6198=DIRECTION('',(0.,0.,1.));
#6199=DIRECTION('',(0.,0.,-1.));
#6200=DIRECTION('center_axis',(0.,1.,0.));
#6201=DIRECTION('ref_axis',(0.70710678118654,0.,0.707106781186555));
#6202=DIRECTION('',(0.,-1.,0.));
#6203=DIRECTION('',(0.,1.,0.));
#6204=DIRECTION('center_axis',(1.,0.,0.));
#6205=DIRECTION('ref_axis',(0.,-0.707106781186546,0.707106781186549));
#6206=DIRECTION('',(-1.,0.,0.));
#6207=DIRECTION('',(1.,0.,0.));
#6208=DIRECTION('center_axis',(0.,-1.,0.));
#6209=DIRECTION('ref_axis',(-0.70710678118654,0.,0.707106781186555));
#6210=DIRECTION('',(0.,1.,0.));
#6211=DIRECTION('',(0.,-1.,0.));
#6212=DIRECTION('center_axis',(-1.,0.,0.));
#6213=DIRECTION('ref_axis',(0.,-0.707106781186546,-0.707106781186549));
#6214=DIRECTION('',(1.,0.,0.));
#6215=DIRECTION('',(-1.,0.,0.));
#6216=DIRECTION('center_axis',(0.,-1.,0.));
#6217=DIRECTION('ref_axis',(0.70710678118654,0.,-0.707106781186555));
#6218=DIRECTION('',(0.,1.,0.));
#6219=DIRECTION('',(0.,-1.,0.));
#6220=DIRECTION('center_axis',(1.,0.,0.));
#6221=DIRECTION('ref_axis',(0.,0.707106781186546,-0.707106781186549));
#6222=DIRECTION('',(-1.,0.,0.));
#6223=DIRECTION('',(1.,0.,0.));
#6224=DIRECTION('center_axis',(0.,1.,0.));
#6225=DIRECTION('ref_axis',(-0.70710678118654,0.,-0.707106781186555));
#6226=DIRECTION('',(0.,-1.,0.));
#6227=DIRECTION('',(0.,1.,0.));
#6228=DIRECTION('center_axis',(-1.,0.,0.));
#6229=DIRECTION('ref_axis',(0.,-1.,0.));
#6230=DIRECTION('center_axis',(1.,0.,0.));
#6231=DIRECTION('ref_axis',(0.,1.,0.));
#6232=DIRECTION('center_axis',(1.,0.,0.));
#6233=DIRECTION('ref_axis',(0.,1.,0.));
#6234=DIRECTION('center_axis',(0.,1.,0.));
#6235=DIRECTION('ref_axis',(-1.,0.,0.));
#6236=DIRECTION('center_axis',(0.,0.,1.));
#6237=DIRECTION('ref_axis',(1.,0.,0.));
#6238=DIRECTION('center_axis',(0.,-1.,0.));
#6239=DIRECTION('ref_axis',(1.,0.,0.));
#6240=DIRECTION('center_axis',(1.,0.,0.));
#6241=DIRECTION('ref_axis',(0.,1.,0.));
#6242=DIRECTION('center_axis',(0.,0.,-1.));
#6243=DIRECTION('ref_axis',(-1.,0.,0.));
#6244=DIRECTION('center_axis',(1.,0.,0.));
#6245=DIRECTION('ref_axis',(0.,1.,0.));
#6246=DIRECTION('',(1.,0.,0.));
#6247=DIRECTION('center_axis',(1.,0.,0.));
#6248=DIRECTION('ref_axis',(0.,1.,0.));
#6249=DIRECTION('center_axis',(1.,0.,0.));
#6250=DIRECTION('ref_axis',(0.,1.,0.));
#6251=DIRECTION('center_axis',(1.,0.,0.));
#6252=DIRECTION('ref_axis',(0.,1.,0.));
#6253=DIRECTION('',(1.,0.,0.));
#6254=DIRECTION('center_axis',(1.,0.,0.));
#6255=DIRECTION('ref_axis',(0.,1.,0.));
#6256=DIRECTION('center_axis',(1.,0.,0.));
#6257=DIRECTION('ref_axis',(0.,1.,0.));
#7663=CARTESIAN_POINT('',(0.,0.,0.));
#7664=CARTESIAN_POINT('Origin',(140.,37.8343839603864,-8.00000000000001));
#7665=CARTESIAN_POINT('',(140.,31.8343839603864,-8.00000000000001));
#7666=CARTESIAN_POINT('Origin',(140.,37.8343839603864,-8.00000000000001));
#7667=CARTESIAN_POINT('',(120.,31.8343839603864,-8.00000000000001));
#7668=CARTESIAN_POINT('',(140.,31.8343839603864,-8.00000000000001));
#7669=CARTESIAN_POINT('Origin',(120.,37.8343839603864,-8.00000000000001));
#7670=CARTESIAN_POINT('Origin',(140.,37.8343839603864,-8.00000000000001));
#7671=CARTESIAN_POINT('',(140.,34.8343839603864,-8.00000000000001));
#7672=CARTESIAN_POINT('Origin',(140.,37.8343839603864,-8.00000000000001));
#7673=CARTESIAN_POINT('Origin',(130.,23.6740181268338,20.));
#7674=CARTESIAN_POINT('',(126.,23.6740181268338,20.));
#7675=CARTESIAN_POINT('Origin',(130.,23.6740181268338,20.));
#7676=CARTESIAN_POINT('',(126.,23.6740181268338,-3.));
#7677=CARTESIAN_POINT('',(126.,23.6740181268338,20.));
#7678=CARTESIAN_POINT('Origin',(130.,23.6740181268338,-3.));
#7679=CARTESIAN_POINT('Origin',(130.,23.6740181268338,-3.));
#7680=CARTESIAN_POINT('Origin',(130.,-23.6740181268338,20.));
#7681=CARTESIAN_POINT('',(126.,-23.6740181268338,20.));
#7682=CARTESIAN_POINT('Origin',(130.,-23.6740181268338,20.));
#7683=CARTESIAN_POINT('',(126.,-23.6740181268338,-3.));
#7684=CARTESIAN_POINT('',(126.,-23.6740181268338,20.));
#7685=CARTESIAN_POINT('Origin',(130.,-23.6740181268338,-3.));
#7686=CARTESIAN_POINT('Origin',(130.,-23.6740181268338,-3.));
#7687=CARTESIAN_POINT('Origin',(150.,-37.8343839603864,-8.00000000000001));
#7688=CARTESIAN_POINT('',(150.,-42.8343839603862,-8.00000000000001));
#7689=CARTESIAN_POINT('Origin',(150.,-37.8343839603864,-8.00000000000001));
#7690=CARTESIAN_POINT('',(142.,-42.8343839603862,-8.00000000000001));
#7691=CARTESIAN_POINT('',(150.,-42.8343839603862,-8.00000000000001));
#7692=CARTESIAN_POINT('Origin',(142.,-37.8343839603864,-8.00000000000001));
#7693=CARTESIAN_POINT('Origin',(142.,-37.8343839603864,-8.00000000000001));
#7694=CARTESIAN_POINT('',(142.,-40.8343839603864,-8.00000000000001));
#7695=CARTESIAN_POINT('Origin',(142.,-37.8343839603864,-8.00000000000001));
#7696=CARTESIAN_POINT('Origin',(150.,37.8343839603864,-8.00000000000001));
#7697=CARTESIAN_POINT('',(150.,32.8343839603866,-8.00000000000001));
#7698=CARTESIAN_POINT('Origin',(150.,37.8343839603864,-8.00000000000001));
#7699=CARTESIAN_POINT('',(142.,32.8343839603866,-8.00000000000001));
#7700=CARTESIAN_POINT('',(150.,32.8343839603866,-8.00000000000001));
#7701=CARTESIAN_POINT('Origin',(142.,37.8343839603864,-8.00000000000001));
#7702=CARTESIAN_POINT('Origin',(142.,37.8343839603864,-8.00000000000001));
#7703=CARTESIAN_POINT('',(142.,34.8343839603864,-8.00000000000001));
#7704=CARTESIAN_POINT('Origin',(142.,37.8343839603864,-8.00000000000001));
#7705=CARTESIAN_POINT('Origin',(150.,37.8343839603864,-8.00000000000001));
#7706=CARTESIAN_POINT('',(150.,34.8343839603864,-8.00000000000001));
#7707=CARTESIAN_POINT('Origin',(150.,-37.8343839603864,-8.00000000000001));
#7708=CARTESIAN_POINT('',(140.,-40.8343839603864,-8.00000000000001));
#7709=CARTESIAN_POINT('',(150.,-40.8343839603864,-8.00000000000001));
#7710=CARTESIAN_POINT('Origin',(140.,-37.8343839603864,-8.00000000000001));
#7711=CARTESIAN_POINT('Origin',(121.,49.,-19.));
#7712=CARTESIAN_POINT('',(120.,49.,-19.));
#7713=CARTESIAN_POINT('',(121.,49.,-20.));
#7714=CARTESIAN_POINT('Origin',(121.,49.,-19.));
#7715=CARTESIAN_POINT('',(121.,50.,-19.));
#7716=CARTESIAN_POINT('Origin',(121.,49.,-19.));
#7717=CARTESIAN_POINT('Origin',(121.,49.,-19.));
#7718=CARTESIAN_POINT('Origin',(121.,-49.,-19.));
#7719=CARTESIAN_POINT('',(121.,-50.,-19.));
#7720=CARTESIAN_POINT('',(121.,-49.,-20.));
#7721=CARTESIAN_POINT('Origin',(121.,-49.,-19.));
#7722=CARTESIAN_POINT('',(120.,-49.,-19.));
#7723=CARTESIAN_POINT('Origin',(121.,-49.,-19.));
#7724=CARTESIAN_POINT('Origin',(121.,-49.,-19.));
#7725=CARTESIAN_POINT('Origin',(149.,49.,-19.));
#7726=CARTESIAN_POINT('',(149.,50.,-19.));
#7727=CARTESIAN_POINT('',(149.,49.,-20.));
#7728=CARTESIAN_POINT('Origin',(149.,49.,-19.));
#7729=CARTESIAN_POINT('',(150.,49.,-19.));
#7730=CARTESIAN_POINT('Origin',(149.,49.,-19.));
#7731=CARTESIAN_POINT('Origin',(149.,49.,-19.));
#7732=CARTESIAN_POINT('Origin',(121.,49.,19.));
#7733=CARTESIAN_POINT('',(121.,50.,19.));
#7734=CARTESIAN_POINT('',(121.,49.,20.));
#7735=CARTESIAN_POINT('Origin',(121.,49.,19.));
#7736=CARTESIAN_POINT('',(120.,49.,19.));
#7737=CARTESIAN_POINT('Origin',(121.,49.,19.));
#7738=CARTESIAN_POINT('Origin',(121.,49.,19.));
#7739=CARTESIAN_POINT('Origin',(121.,49.,0.));
#7740=CARTESIAN_POINT('',(121.,50.,0.));
#7741=CARTESIAN_POINT('',(120.,49.,0.));
#7742=CARTESIAN_POINT('Origin',(149.,-49.,-19.));
#7743=CARTESIAN_POINT('',(150.,-49.,-19.));
#7744=CARTESIAN_POINT('',(149.,-49.,-20.));
#7745=CARTESIAN_POINT('Origin',(149.,-49.,-19.));
#7746=CARTESIAN_POINT('',(149.,-50.,-19.));
#7747=CARTESIAN_POINT('Origin',(149.,-49.,-19.));
#7748=CARTESIAN_POINT('Origin',(149.,-49.,-19.));
#7749=CARTESIAN_POINT('Origin',(121.,-49.,19.));
#7750=CARTESIAN_POINT('',(120.,-49.,19.));
#7751=CARTESIAN_POINT('',(121.,-49.,20.));
#7752=CARTESIAN_POINT('Origin',(121.,-49.,19.));
#7753=CARTESIAN_POINT('',(121.,-50.,19.));
#7754=CARTESIAN_POINT('Origin',(121.,-49.,19.));
#7755=CARTESIAN_POINT('Origin',(121.,-49.,19.));
#7756=CARTESIAN_POINT('Origin',(121.,-49.,0.));
#7757=CARTESIAN_POINT('',(120.,-49.,0.));
#7758=CARTESIAN_POINT('',(121.,-50.,0.));
#7759=CARTESIAN_POINT('Origin',(149.,49.,19.));
#7760=CARTESIAN_POINT('',(150.,49.,19.));
#7761=CARTESIAN_POINT('',(149.,49.,20.));
#7762=CARTESIAN_POINT('Origin',(149.,49.,19.));
#7763=CARTESIAN_POINT('',(149.,50.,19.));
#7764=CARTESIAN_POINT('Origin',(149.,49.,19.));
#7765=CARTESIAN_POINT('Origin',(149.,49.,19.));
#7766=CARTESIAN_POINT('Origin',(149.,49.,0.));
#7767=CARTESIAN_POINT('',(150.,49.,0.));
#7768=CARTESIAN_POINT('',(149.,50.,0.));
#7769=CARTESIAN_POINT('Origin',(142.5,49.,19.));
#7770=CARTESIAN_POINT('',(142.5,49.,20.));
#7771=CARTESIAN_POINT('',(142.5,50.,19.));
#7772=CARTESIAN_POINT('Origin',(149.,-49.,19.));
#7773=CARTESIAN_POINT('',(149.,-50.,19.));
#7774=CARTESIAN_POINT('',(149.,-49.,20.));
#7775=CARTESIAN_POINT('Origin',(149.,-49.,19.));
#7776=CARTESIAN_POINT('',(150.,-49.,19.));
#7777=CARTESIAN_POINT('Origin',(149.,-49.,19.));
#7778=CARTESIAN_POINT('Origin',(149.,-49.,19.));
#7779=CARTESIAN_POINT('Origin',(149.,-49.,0.));
#7780=CARTESIAN_POINT('',(150.,-49.,0.));
#7781=CARTESIAN_POINT('',(149.,-50.,0.));
#7782=CARTESIAN_POINT('Origin',(149.,-25.,19.));
#7783=CARTESIAN_POINT('',(149.,-25.,20.));
#7784=CARTESIAN_POINT('',(150.,-25.,19.));
#7785=CARTESIAN_POINT('Origin',(127.5,-49.,19.));
#7786=CARTESIAN_POINT('',(127.5,-49.,20.));
#7787=CARTESIAN_POINT('',(127.5,-50.,19.));
#7788=CARTESIAN_POINT('Origin',(121.,25.,19.));
#7789=CARTESIAN_POINT('',(121.,25.,20.));
#7790=CARTESIAN_POINT('',(120.,25.,19.));
#7791=CARTESIAN_POINT('Origin',(127.5,-49.,-19.));
#7792=CARTESIAN_POINT('',(127.5,-49.,-20.));
#7793=CARTESIAN_POINT('',(127.5,-50.,-19.));
#7794=CARTESIAN_POINT('Origin',(149.,-25.,-19.));
#7795=CARTESIAN_POINT('',(149.,-25.,-20.));
#7796=CARTESIAN_POINT('',(150.,-25.,-19.));
#7797=CARTESIAN_POINT('Origin',(142.5,49.,-19.));
#7798=CARTESIAN_POINT('',(142.5,49.,-20.));
#7799=CARTESIAN_POINT('',(142.5,50.,-19.));
#7800=CARTESIAN_POINT('Origin',(121.,25.,-19.));
#7801=CARTESIAN_POINT('',(121.,25.,-20.));
#7802=CARTESIAN_POINT('',(120.,25.,-19.));
#7803=CARTESIAN_POINT('Origin',(120.,50.,0.));
#7804=CARTESIAN_POINT('',(120.,-7.50000000000001,9.6119802892091E-15));
#7805=CARTESIAN_POINT('Origin',(120.,1.91963385766348E-15,1.05304653885696E-14));
#7806=CARTESIAN_POINT('',(120.,-43.8343839603864,-7.99999999999999));
#7807=CARTESIAN_POINT('Origin',(120.,-37.8343839603864,-7.99999999999999));
#7808=CARTESIAN_POINT('Origin',(150.,50.,0.));
#7809=CARTESIAN_POINT('Origin',(135.,8.88178419700125E-15,20.));
#7810=CARTESIAN_POINT('Origin',(120.,-50.,0.));
#7811=CARTESIAN_POINT('Origin',(150.,-50.,0.));
#7812=CARTESIAN_POINT('Origin',(135.,8.88178419700125E-15,-20.));
#7813=CARTESIAN_POINT('Origin',(0.,-37.8343839603864,-7.99999999999999));
#7814=CARTESIAN_POINT('',(140.,-43.8343839603864,-7.99999999999999));
#7815=CARTESIAN_POINT('',(0.,-43.8343839603864,-7.99999999999999));
#7816=CARTESIAN_POINT('Origin',(140.,-37.8343839603864,-7.99999999999999));
#7817=CARTESIAN_POINT('Origin',(140.,-37.8343839603864,-7.99999999999999));
#7818=CARTESIAN_POINT('Origin',(0.,1.91963385766348E-15,1.05304653885696E-14));
#7819=CARTESIAN_POINT('',(140.,-7.50000000000001,9.6119802892091E-15));
#7820=CARTESIAN_POINT('',(0.,-7.50000000000001,9.61198028920908E-15));
#7821=CARTESIAN_POINT('Origin',(140.,1.91963385766348E-15,1.05304653885696E-14));
#7822=CARTESIAN_POINT('Origin',(140.,2.22044604925031E-15,9.99200722162641E-15));
#9477=UNCERTAINTY_MEASURE_WITH_UNIT(LENGTH_MEASURE(0.01),#9497,
'DISTANCE_ACCURACY_VALUE',
'Maximum model space distance between geometric entities at asserted c
onnectivities');
#9485=UNCERTAINTY_MEASURE_WITH_UNIT(LENGTH_MEASURE(0.01),#9497,
'DISTANCE_ACCURACY_VALUE',
'Maximum model space distance between geometric entities at asserted c
onnectivities');
#9488=(
GEOMETRIC_REPRESENTATION_CONTEXT(3)
GLOBAL_UNCERTAINTY_ASSIGNED_CONTEXT((#9477))
GLOBAL_UNIT_ASSIGNED_CONTEXT((#9497,#9499,#9500))
REPRESENTATION_CONTEXT('','3D')
);
#9496=(
GEOMETRIC_REPRESENTATION_CONTEXT(3)
GLOBAL_UNCERTAINTY_ASSIGNED_CONTEXT((#9485))
GLOBAL_UNIT_ASSIGNED_CONTEXT((#9497,#9499,#9500))
REPRESENTATION_CONTEXT('','3D')
);
#9497=(
LENGTH_UNIT()
NAMED_UNIT(*)
SI_UNIT(.MILLI.,.METRE.)
);
#9499=(
NAMED_UNIT(*)
PLANE_ANGLE_UNIT()
SI_UNIT($,.RADIAN.)
);
#9500=(
NAMED_UNIT(*)
SI_UNIT($,.STERADIAN.)
SOLID_ANGLE_UNIT()
);
#9503=SHAPE_DEFINITION_REPRESENTATION(#9513,#9540);
#9513=PRODUCT_DEFINITION_SHAPE('',$,#9551);
#9540=SHAPE_REPRESENTATION('',(#5213),#9488);
#9548=PRODUCT_DEFINITION_CONTEXT('part definition',#9580,'design');
#9551=PRODUCT_DEFINITION('End_plates','End_plates',#9561,#9548);
#9561=PRODUCT_DEFINITION_FORMATION('',$,#9584);
#9580=APPLICATION_CONTEXT(
'Core Data for Automotive Mechanical Design Process');
#9581=PRODUCT_CONTEXT('part definition',#9580,'mechanical');
#9584=PRODUCT('End_plates','End_plates',$,(#9581));
#9593=PRESENTATION_STYLE_ASSIGNMENT((#9596));
#9596=SURFACE_STYLE_USAGE(.BOTH.,#9599);
#9599=SURFACE_SIDE_STYLE('',(#9602));
#9602=SURFACE_STYLE_FILL_AREA(#9605);
#9605=FILL_AREA_STYLE('Opaque(245,245,246)',(#9608));
#9608=FILL_AREA_STYLE_COLOUR('Opaque(245,245,246)',#9611);
#9611=COLOUR_RGB('Opaque(245,245,246)', 0.66274510, 0.83137255, 0.94901961);
ENDSEC;
END-ISO-10303-21;
